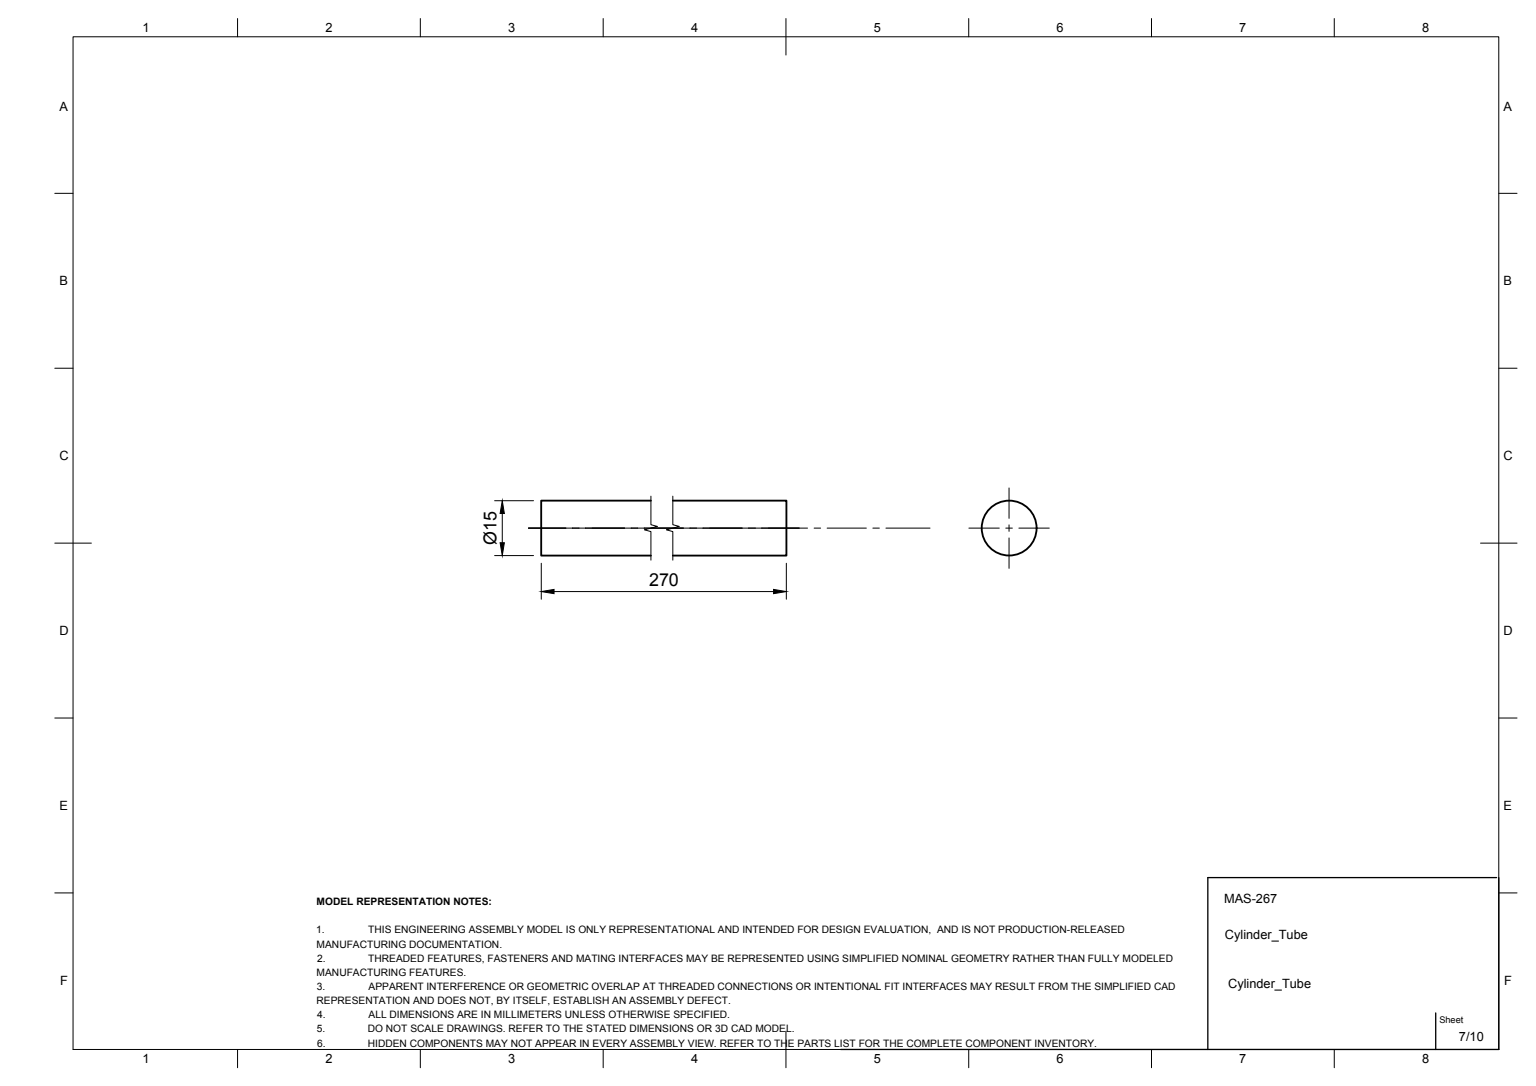
ISO-10303-21;
HEADER;
/* Generated by software containing ST-Developer
 * from STEP Tools, Inc. (www.steptools.com) 
 */

FILE_DESCRIPTION(
/* description */ (''),
/* implementation_level */ '2;1');

FILE_NAME(
/* name */ 'Cylinder_Tube.step',
/* time_stamp */ '2026-10-12T15:29:24-07:00',
/* author */ (''),
/* organization */ (''),
/* preprocessor_version */ 'ST-DEVELOPER v20.2',
/* originating_system */ 'Autodesk Translation Framework v15.15.0.0',
/* authorisation */ '');

FILE_SCHEMA (('AUTOMOTIVE_DESIGN { 1 0 10303 214 3 1 1 }'));
ENDSEC;

DATA;
#10=MECHANICAL_DESIGN_GEOMETRIC_PRESENTATION_REPRESENTATION('',(#196),#9496);
#150=SHAPE_REPRESENTATION_RELATIONSHIP('SRR','None',#9544,#159);
#159=ADVANCED_BREP_SHAPE_REPRESENTATION('',(#253),#9492);
#196=STYLED_ITEM('',(#9594),#253);
#253=MANIFOLD_SOLID_BREP('Body1',#4998);
#564=PLANE('',#5557);
#565=PLANE('',#5561);
#831=FACE_OUTER_BOUND('',#1246,.T.);
#832=FACE_OUTER_BOUND('',#1247,.T.);
#833=FACE_OUTER_BOUND('',#1248,.T.);
#1246=EDGE_LOOP('',(#4047));
#1247=EDGE_LOOP('',(#4048,#4049,#4050,#4051));
#1248=EDGE_LOOP('',(#4052));
#1565=LINE('',#8625,#1802);
#1802=VECTOR('',#6834,7.50000000000001);
#2138=CIRCLE('',#5558,7.50000000000001);
#2139=CIRCLE('',#5560,7.50000000000001);
#2523=VERTEX_POINT('',#8620);
#2524=VERTEX_POINT('',#8623);
#3076=EDGE_CURVE('',#2523,#2523,#2138,.T.);
#3077=EDGE_CURVE('',#2524,#2524,#2139,.T.);
#3078=EDGE_CURVE('',#2524,#2523,#1565,.T.);
#4047=ORIENTED_EDGE('',*,*,#3076,.T.);
#4048=ORIENTED_EDGE('',*,*,#3077,.F.);
#4049=ORIENTED_EDGE('',*,*,#3078,.T.);
#4050=ORIENTED_EDGE('',*,*,#3076,.F.);
#4051=ORIENTED_EDGE('',*,*,#3078,.F.);
#4052=ORIENTED_EDGE('',*,*,#3077,.T.);
#4606=CYLINDRICAL_SURFACE('',#5559,7.50000000000001);
#4842=ADVANCED_FACE('',(#831),#564,.F.);
#4843=ADVANCED_FACE('',(#832),#4606,.T.);
#4844=ADVANCED_FACE('',(#833),#565,.T.);
#4998=CLOSED_SHELL('',(#4842,#4843,#4844));
#5556=AXIS2_PLACEMENT_3D('',#8618,#6824,#6825);
#5557=AXIS2_PLACEMENT_3D('',#8619,#6826,#6827);
#5558=AXIS2_PLACEMENT_3D('',#8621,#6828,#6829);
#5559=AXIS2_PLACEMENT_3D('',#8622,#6830,#6831);
#5560=AXIS2_PLACEMENT_3D('',#8624,#6832,#6833);
#5561=AXIS2_PLACEMENT_3D('',#8626,#6835,#6836);
#6824=DIRECTION('axis',(0.,0.,1.));
#6825=DIRECTION('refdir',(1.,0.,0.));
#6826=DIRECTION('center_axis',(1.,0.,0.));
#6827=DIRECTION('ref_axis',(0.,1.,0.));
#6828=DIRECTION('center_axis',(-1.,0.,0.));
#6829=DIRECTION('ref_axis',(0.,1.,0.));
#6830=DIRECTION('center_axis',(1.,0.,0.));
#6831=DIRECTION('ref_axis',(0.,1.,0.));
#6832=DIRECTION('center_axis',(1.,0.,0.));
#6833=DIRECTION('ref_axis',(0.,1.,0.));
#6834=DIRECTION('',(-1.,0.,0.));
#6835=DIRECTION('center_axis',(1.,0.,0.));
#6836=DIRECTION('ref_axis',(0.,1.,0.));
#8618=CARTESIAN_POINT('',(0.,0.,0.));
#8619=CARTESIAN_POINT('Origin',(-135.,2.22044604925031E-15,9.99200722162641E-15));
#8620=CARTESIAN_POINT('',(-135.,-7.50000000000001,9.6119802892091E-15));
#8621=CARTESIAN_POINT('Origin',(-135.,1.91963385766348E-15,1.05304653885696E-14));
#8622=CARTESIAN_POINT('Origin',(0.,1.91963385766348E-15,1.05304653885696E-14));
#8623=CARTESIAN_POINT('',(135.,-7.50000000000001,9.6119802892091E-15));
#8624=CARTESIAN_POINT('Origin',(135.,1.91963385766348E-15,1.05304653885696E-14));
#8625=CARTESIAN_POINT('',(0.,-7.50000000000001,9.61198028920908E-15));
#8626=CARTESIAN_POINT('Origin',(135.,2.22044604925031E-15,9.99200722162641E-15));
#9481=UNCERTAINTY_MEASURE_WITH_UNIT(LENGTH_MEASURE(0.01),#9497,
'DISTANCE_ACCURACY_VALUE',
'Maximum model space distance between geometric entities at asserted c
onnectivities');
#9485=UNCERTAINTY_MEASURE_WITH_UNIT(LENGTH_MEASURE(0.01),#9497,
'DISTANCE_ACCURACY_VALUE',
'Maximum model space distance between geometric entities at asserted c
onnectivities');
#9492=(
GEOMETRIC_REPRESENTATION_CONTEXT(3)
GLOBAL_UNCERTAINTY_ASSIGNED_CONTEXT((#9481))
GLOBAL_UNIT_ASSIGNED_CONTEXT((#9497,#9499,#9500))
REPRESENTATION_CONTEXT('','3D')
);
#9496=(
GEOMETRIC_REPRESENTATION_CONTEXT(3)
GLOBAL_UNCERTAINTY_ASSIGNED_CONTEXT((#9485))
GLOBAL_UNIT_ASSIGNED_CONTEXT((#9497,#9499,#9500))
REPRESENTATION_CONTEXT('','3D')
);
#9497=(
LENGTH_UNIT()
NAMED_UNIT(*)
SI_UNIT(.MILLI.,.METRE.)
);
#9499=(
NAMED_UNIT(*)
PLANE_ANGLE_UNIT()
SI_UNIT($,.RADIAN.)
);
#9500=(
NAMED_UNIT(*)
SI_UNIT($,.STERADIAN.)
SOLID_ANGLE_UNIT()
);
#9507=SHAPE_DEFINITION_REPRESENTATION(#9517,#9544);
#9517=PRODUCT_DEFINITION_SHAPE('',$,#9555);
#9544=SHAPE_REPRESENTATION('',(#5556),#9492);
#9548=PRODUCT_DEFINITION_CONTEXT('part definition',#9580,'design');
#9555=PRODUCT_DEFINITION('Cylinder_Tube','Cylinder_Tube',#9565,#9548);
#9565=PRODUCT_DEFINITION_FORMATION('',$,#9588);
#9580=APPLICATION_CONTEXT(
'Core Data for Automotive Mechanical Design Process');
#9581=PRODUCT_CONTEXT('part definition',#9580,'mechanical');
#9588=PRODUCT('Cylinder_Tube','Cylinder_Tube',$,(#9581));
#9594=PRESENTATION_STYLE_ASSIGNMENT((#9597));
#9597=SURFACE_STYLE_USAGE(.BOTH.,#9600);
#9600=SURFACE_SIDE_STYLE('',(#9603));
#9603=SURFACE_STYLE_FILL_AREA(#9606);
#9606=FILL_AREA_STYLE('Opaque(160,160,160)',(#9609));
#9609=FILL_AREA_STYLE_COLOUR('Opaque(160,160,160)',#9612);
#9612=COLOUR_RGB('Opaque(160,160,160)', 0.40784314, 0.44705882, 0.49803922);
ENDSEC;
END-ISO-10303-21;
